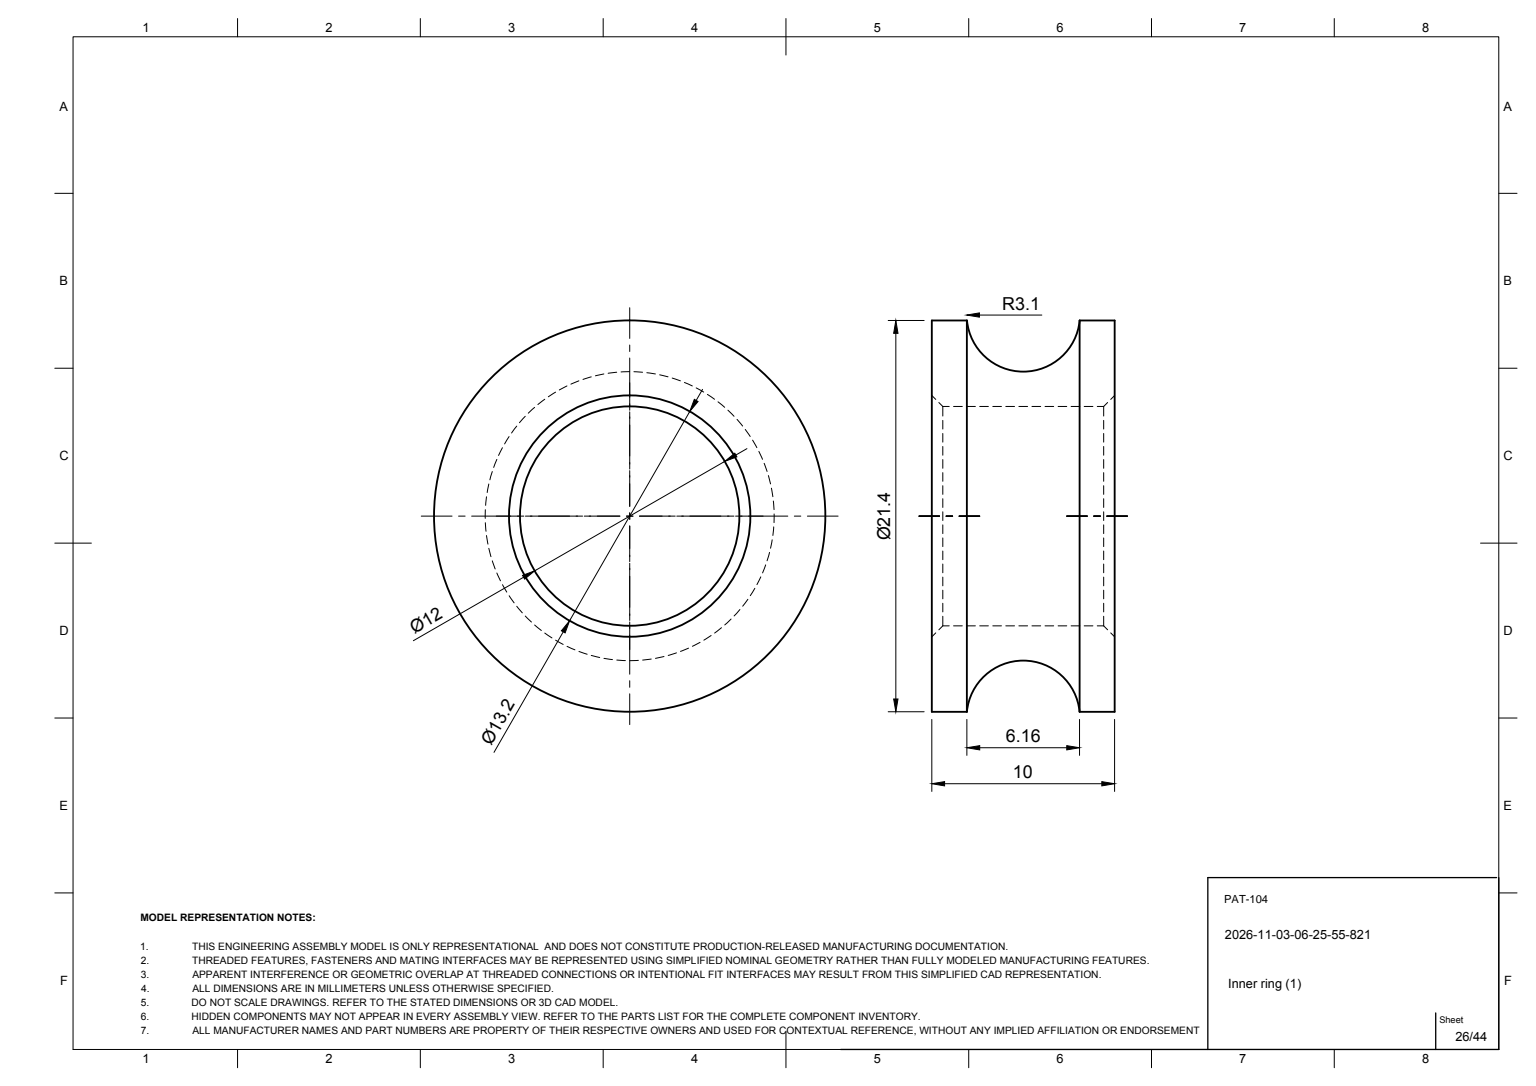
ISO-10303-21;
HEADER;
/* Generated by software containing ST-Developer
 * from STEP Tools, Inc. (www.steptools.com) 
 */

FILE_DESCRIPTION(
/* description */ ('Timing belt drive module 2 mm Pitch Timing 20T-40T'),

/* implementation_level */ '2;1');

FILE_NAME(
/* name */ 'Inner ring (1).step',
/* time_stamp */ '2026-10-28T03:25:12-07:00',
/* author */ (''),
/* organization */ (''),
/* preprocessor_version */ 'ST-DEVELOPER v20.2',
/* originating_system */ 'Autodesk Translation Framework v15.17.0.0',
/* authorisation */ '');

FILE_SCHEMA (('AUTOMOTIVE_DESIGN { 1 0 10303 214 3 1 1 }'));
ENDSEC;

DATA;
#10=MECHANICAL_DESIGN_GEOMETRIC_PRESENTATION_REPRESENTATION('',(#554),#17830);
#423=CONICAL_SURFACE('',#10053,0.63,0.785398163397448);
#424=CONICAL_SURFACE('',#10060,0.63,0.785398163397448);
#436=TOROIDAL_SURFACE('',#10042,1.1,0.309556);
#460=SHAPE_REPRESENTATION_RELATIONSHIP('SRR','None',#18032,#503);
#503=ADVANCED_BREP_SHAPE_REPRESENTATION('',(#611),#17807);
#554=STYLED_ITEM('',(#18317),#611);
#611=MANIFOLD_SOLID_BREP('Body1',#9012);
#720=FACE_BOUND('',#1807,.T.);
#721=FACE_BOUND('',#1810,.T.);
#882=PLANE('',#10055);
#883=PLANE('',#10058);
#1198=FACE_OUTER_BOUND('',#1802,.T.);
#1199=FACE_OUTER_BOUND('',#1803,.T.);
#1200=FACE_OUTER_BOUND('',#1804,.T.);
#1201=FACE_OUTER_BOUND('',#1805,.T.);
#1202=FACE_OUTER_BOUND('',#1806,.T.);
#1203=FACE_OUTER_BOUND('',#1808,.T.);
#1204=FACE_OUTER_BOUND('',#1809,.T.);
#1205=FACE_OUTER_BOUND('',#1811,.T.);
#1802=EDGE_LOOP('',(#6823,#6824,#6825,#6826,#6827,#6828));
#1803=EDGE_LOOP('',(#6829,#6830,#6831,#6832,#6833));
#1804=EDGE_LOOP('',(#6834,#6835,#6836,#6837));
#1805=EDGE_LOOP('',(#6838,#6839,#6840,#6841));
#1806=EDGE_LOOP('',(#6842));
#1807=EDGE_LOOP('',(#6843));
#1808=EDGE_LOOP('',(#6844,#6845,#6846,#6847,#6848));
#1809=EDGE_LOOP('',(#6849));
#1810=EDGE_LOOP('',(#6850));
#1811=EDGE_LOOP('',(#6851,#6852,#6853,#6854));
#2398=CIRCLE('',#10043,1.070235);
#2399=CIRCLE('',#10044,1.070235);
#2400=CIRCLE('',#10045,0.309556);
#2401=CIRCLE('',#10046,1.070235);
#2402=CIRCLE('',#10047,1.070235);
#2403=CIRCLE('',#10049,1.070235);
#2404=CIRCLE('',#10051,0.6);
#2405=CIRCLE('',#10052,0.6);
#2406=CIRCLE('',#10054,0.66);
#2407=CIRCLE('',#10057,1.070235);
#2408=CIRCLE('',#10059,0.66);
#3039=LINE('',#15374,#3517);
#3040=LINE('',#15380,#3518);
#3041=LINE('',#15384,#3519);
#3042=LINE('',#15390,#3520);
#3043=LINE('',#15395,#3521);
#3517=VECTOR('',#12124,1.070235);
#3518=VECTOR('',#12131,0.6);
#3519=VECTOR('',#12136,0.63);
#3520=VECTOR('',#12145,1.070235);
#3521=VECTOR('',#12152,0.63);
#4104=VERTEX_POINT('',#15363);
#4105=VERTEX_POINT('',#15364);
#4106=VERTEX_POINT('',#15367);
#4107=VERTEX_POINT('',#15369);
#4108=VERTEX_POINT('',#15373);
#4109=VERTEX_POINT('',#15377);
#4110=VERTEX_POINT('',#15379);
#4111=VERTEX_POINT('',#15383);
#4112=VERTEX_POINT('',#15388);
#4113=VERTEX_POINT('',#15392);
#5094=EDGE_CURVE('',#4104,#4105,#2398,.T.);
#5095=EDGE_CURVE('',#4105,#4104,#2399,.T.);
#5096=EDGE_CURVE('',#4105,#4106,#2400,.T.);
#5097=EDGE_CURVE('',#4107,#4106,#2401,.T.);
#5098=EDGE_CURVE('',#4106,#4107,#2402,.T.);
#5099=EDGE_CURVE('',#4107,#4108,#3039,.T.);
#5100=EDGE_CURVE('',#4108,#4108,#2403,.T.);
#5101=EDGE_CURVE('',#4109,#4109,#2404,.T.);
#5102=EDGE_CURVE('',#4109,#4110,#3040,.T.);
#5103=EDGE_CURVE('',#4110,#4110,#2405,.T.);
#5104=EDGE_CURVE('',#4110,#4111,#3041,.T.);
#5105=EDGE_CURVE('',#4111,#4111,#2406,.T.);
#5106=EDGE_CURVE('',#4112,#4112,#2407,.T.);
#5107=EDGE_CURVE('',#4112,#4104,#3042,.T.);
#5108=EDGE_CURVE('',#4113,#4113,#2408,.T.);
#5109=EDGE_CURVE('',#4113,#4109,#3043,.T.);
#6823=ORIENTED_EDGE('',*,*,#5094,.F.);
#6824=ORIENTED_EDGE('',*,*,#5095,.F.);
#6825=ORIENTED_EDGE('',*,*,#5096,.T.);
#6826=ORIENTED_EDGE('',*,*,#5097,.F.);
#6827=ORIENTED_EDGE('',*,*,#5098,.F.);
#6828=ORIENTED_EDGE('',*,*,#5096,.F.);
#6829=ORIENTED_EDGE('',*,*,#5097,.T.);
#6830=ORIENTED_EDGE('',*,*,#5098,.T.);
#6831=ORIENTED_EDGE('',*,*,#5099,.T.);
#6832=ORIENTED_EDGE('',*,*,#5100,.T.);
#6833=ORIENTED_EDGE('',*,*,#5099,.F.);
#6834=ORIENTED_EDGE('',*,*,#5101,.T.);
#6835=ORIENTED_EDGE('',*,*,#5102,.T.);
#6836=ORIENTED_EDGE('',*,*,#5103,.F.);
#6837=ORIENTED_EDGE('',*,*,#5102,.F.);
#6838=ORIENTED_EDGE('',*,*,#5103,.T.);
#6839=ORIENTED_EDGE('',*,*,#5104,.T.);
#6840=ORIENTED_EDGE('',*,*,#5105,.F.);
#6841=ORIENTED_EDGE('',*,*,#5104,.F.);
#6842=ORIENTED_EDGE('',*,*,#5100,.F.);
#6843=ORIENTED_EDGE('',*,*,#5105,.T.);
#6844=ORIENTED_EDGE('',*,*,#5106,.F.);
#6845=ORIENTED_EDGE('',*,*,#5107,.T.);
#6846=ORIENTED_EDGE('',*,*,#5094,.T.);
#6847=ORIENTED_EDGE('',*,*,#5095,.T.);
#6848=ORIENTED_EDGE('',*,*,#5107,.F.);
#6849=ORIENTED_EDGE('',*,*,#5106,.T.);
#6850=ORIENTED_EDGE('',*,*,#5108,.F.);
#6851=ORIENTED_EDGE('',*,*,#5108,.T.);
#6852=ORIENTED_EDGE('',*,*,#5109,.T.);
#6853=ORIENTED_EDGE('',*,*,#5101,.F.);
#6854=ORIENTED_EDGE('',*,*,#5109,.F.);
#8282=CYLINDRICAL_SURFACE('',#10048,1.070235);
#8283=CYLINDRICAL_SURFACE('',#10050,0.6);
#8284=CYLINDRICAL_SURFACE('',#10056,1.070235);
#8696=ADVANCED_FACE('',(#1198),#436,.F.);
#8697=ADVANCED_FACE('',(#1199),#8282,.T.);
#8698=ADVANCED_FACE('',(#1200),#8283,.F.);
#8699=ADVANCED_FACE('',(#1201),#423,.F.);
#8700=ADVANCED_FACE('',(#1202,#720),#882,.T.);
#8701=ADVANCED_FACE('',(#1203),#8284,.T.);
#8702=ADVANCED_FACE('',(#1204,#721),#883,.T.);
#8703=ADVANCED_FACE('',(#1205),#424,.F.);
#9012=CLOSED_SHELL('',(#8696,#8697,#8698,#8699,#8700,#8701,#8702,#8703));
#10041=AXIS2_PLACEMENT_3D('',#15361,#12108,#12109);
#10042=AXIS2_PLACEMENT_3D('',#15362,#12110,#12111);
#10043=AXIS2_PLACEMENT_3D('',#15365,#12112,#12113);
#10044=AXIS2_PLACEMENT_3D('',#15366,#12114,#12115);
#10045=AXIS2_PLACEMENT_3D('',#15368,#12116,#12117);
#10046=AXIS2_PLACEMENT_3D('',#15370,#12118,#12119);
#10047=AXIS2_PLACEMENT_3D('',#15371,#12120,#12121);
#10048=AXIS2_PLACEMENT_3D('',#15372,#12122,#12123);
#10049=AXIS2_PLACEMENT_3D('',#15375,#12125,#12126);
#10050=AXIS2_PLACEMENT_3D('',#15376,#12127,#12128);
#10051=AXIS2_PLACEMENT_3D('',#15378,#12129,#12130);
#10052=AXIS2_PLACEMENT_3D('',#15381,#12132,#12133);
#10053=AXIS2_PLACEMENT_3D('',#15382,#12134,#12135);
#10054=AXIS2_PLACEMENT_3D('',#15385,#12137,#12138);
#10055=AXIS2_PLACEMENT_3D('',#15386,#12139,#12140);
#10056=AXIS2_PLACEMENT_3D('',#15387,#12141,#12142);
#10057=AXIS2_PLACEMENT_3D('',#15389,#12143,#12144);
#10058=AXIS2_PLACEMENT_3D('',#15391,#12146,#12147);
#10059=AXIS2_PLACEMENT_3D('',#15393,#12148,#12149);
#10060=AXIS2_PLACEMENT_3D('',#15394,#12150,#12151);
#12108=DIRECTION('axis',(0.,0.,1.));
#12109=DIRECTION('refdir',(1.,0.,0.));
#12110=DIRECTION('center_axis',(0.,-1.,0.));
#12111=DIRECTION('ref_axis',(0.,0.,-1.));
#12112=DIRECTION('center_axis',(0.,-1.,0.));
#12113=DIRECTION('ref_axis',(1.,0.,0.));
#12114=DIRECTION('center_axis',(0.,-1.,0.));
#12115=DIRECTION('ref_axis',(1.,0.,0.));
#12116=DIRECTION('center_axis',(1.,0.,1.22464679914735E-16));
#12117=DIRECTION('ref_axis',(-1.22464679914735E-16,0.,1.));
#12118=DIRECTION('center_axis',(0.,1.,0.));
#12119=DIRECTION('ref_axis',(1.,0.,0.));
#12120=DIRECTION('center_axis',(0.,1.,0.));
#12121=DIRECTION('ref_axis',(1.,0.,0.));
#12122=DIRECTION('center_axis',(0.,-1.,0.));
#12123=DIRECTION('ref_axis',(1.,0.,0.));
#12124=DIRECTION('',(0.,1.,0.));
#12125=DIRECTION('center_axis',(0.,-1.,0.));
#12126=DIRECTION('ref_axis',(1.,0.,0.));
#12127=DIRECTION('center_axis',(0.,-1.,0.));
#12128=DIRECTION('ref_axis',(1.,0.,0.));
#12129=DIRECTION('center_axis',(0.,-1.,0.));
#12130=DIRECTION('ref_axis',(1.,0.,0.));
#12131=DIRECTION('',(0.,1.,0.));
#12132=DIRECTION('center_axis',(0.,-1.,0.));
#12133=DIRECTION('ref_axis',(1.,0.,0.));
#12134=DIRECTION('center_axis',(0.,1.,0.));
#12135=DIRECTION('ref_axis',(1.,0.,0.));
#12136=DIRECTION('',(-0.707106781186548,0.707106781186547,-8.65956056235493E-17));
#12137=DIRECTION('center_axis',(0.,-1.,0.));
#12138=DIRECTION('ref_axis',(1.,0.,0.));
#12139=DIRECTION('center_axis',(0.,1.,0.));
#12140=DIRECTION('ref_axis',(0.,0.,1.));
#12141=DIRECTION('center_axis',(0.,-1.,0.));
#12142=DIRECTION('ref_axis',(1.,0.,0.));
#12143=DIRECTION('center_axis',(0.,-1.,0.));
#12144=DIRECTION('ref_axis',(1.,0.,0.));
#12145=DIRECTION('',(0.,1.,0.));
#12146=DIRECTION('center_axis',(0.,-1.,0.));
#12147=DIRECTION('ref_axis',(0.,0.,-1.));
#12148=DIRECTION('center_axis',(0.,-1.,0.));
#12149=DIRECTION('ref_axis',(1.,0.,0.));
#12150=DIRECTION('center_axis',(0.,-1.,0.));
#12151=DIRECTION('ref_axis',(1.,0.,0.));
#12152=DIRECTION('',(0.707106781186548,0.707106781186547,8.65956056235493E-17));
#15361=CARTESIAN_POINT('',(0.,0.,0.));
#15362=CARTESIAN_POINT('Origin',(0.,0.,0.));
#15363=CARTESIAN_POINT('',(-1.070235,-0.308121667383195,-1.31065986708547E-16));
#15364=CARTESIAN_POINT('',(-1.31065986708547E-16,-0.308121667383195,1.070235));
#15365=CARTESIAN_POINT('Origin',(0.,-0.308121667383195,0.));
#15366=CARTESIAN_POINT('Origin',(0.,-0.308121667383195,0.));
#15367=CARTESIAN_POINT('',(-1.31065986708547E-16,0.308121667383195,1.070235));
#15368=CARTESIAN_POINT('Origin',(-1.34711147906209E-16,0.,1.1));
#15369=CARTESIAN_POINT('',(-1.070235,0.308121667383195,1.31065986708547E-16));
#15370=CARTESIAN_POINT('Origin',(0.,0.308121667383195,0.));
#15371=CARTESIAN_POINT('Origin',(0.,0.308121667383195,0.));
#15372=CARTESIAN_POINT('Origin',(0.,0.,0.));
#15373=CARTESIAN_POINT('',(-1.070235,0.5,-1.31065986708547E-16));
#15374=CARTESIAN_POINT('',(-1.070235,0.,-1.31065986708547E-16));
#15375=CARTESIAN_POINT('Origin',(0.,0.5,0.));
#15376=CARTESIAN_POINT('Origin',(0.,0.,0.));
#15377=CARTESIAN_POINT('',(-0.6,-0.44,-7.34788079488412E-17));
#15378=CARTESIAN_POINT('Origin',(0.,-0.44,0.));
#15379=CARTESIAN_POINT('',(-0.6,0.44,-7.34788079488412E-17));
#15380=CARTESIAN_POINT('',(-0.6,0.,-7.34788079488412E-17));
#15381=CARTESIAN_POINT('Origin',(0.,0.44,0.));
#15382=CARTESIAN_POINT('Origin',(0.,0.47,0.));
#15383=CARTESIAN_POINT('',(-0.66,0.5,-8.08266887437253E-17));
#15384=CARTESIAN_POINT('',(-0.63,0.47,-7.71527483462832E-17));
#15385=CARTESIAN_POINT('Origin',(0.,0.5,0.));
#15386=CARTESIAN_POINT('Origin',(1.070235,0.5,0.));
#15387=CARTESIAN_POINT('Origin',(0.,0.,0.));
#15388=CARTESIAN_POINT('',(-1.070235,-0.5,-1.31065986708547E-16));
#15389=CARTESIAN_POINT('Origin',(0.,-0.5,0.));
#15390=CARTESIAN_POINT('',(-1.070235,0.,-1.31065986708547E-16));
#15391=CARTESIAN_POINT('Origin',(0.66,-0.5,0.));
#15392=CARTESIAN_POINT('',(-0.66,-0.5,-8.08266887437253E-17));
#15393=CARTESIAN_POINT('Origin',(0.,-0.5,0.));
#15394=CARTESIAN_POINT('Origin',(0.,-0.47,0.));
#15395=CARTESIAN_POINT('',(-0.63,-0.47,-7.71527483462832E-17));
#17757=UNCERTAINTY_MEASURE_WITH_UNIT(LENGTH_MEASURE(0.001),#17831,
'DISTANCE_ACCURACY_VALUE',
'Maximum model space distance between geometric entities at asserted c
onnectivities');
#17780=UNCERTAINTY_MEASURE_WITH_UNIT(LENGTH_MEASURE(0.001),#17831,
'DISTANCE_ACCURACY_VALUE',
'Maximum model space distance between geometric entities at asserted c
onnectivities');
#17807=(
GEOMETRIC_REPRESENTATION_CONTEXT(3)
GLOBAL_UNCERTAINTY_ASSIGNED_CONTEXT((#17757))
GLOBAL_UNIT_ASSIGNED_CONTEXT((#17831,#17833,#17834))
REPRESENTATION_CONTEXT('','3D')
);
#17830=(
GEOMETRIC_REPRESENTATION_CONTEXT(3)
GLOBAL_UNCERTAINTY_ASSIGNED_CONTEXT((#17780))
GLOBAL_UNIT_ASSIGNED_CONTEXT((#17831,#17833,#17834))
REPRESENTATION_CONTEXT('','3D')
);
#17831=(
LENGTH_UNIT()
NAMED_UNIT(*)
SI_UNIT(.CENTI.,.METRE.)
);
#17833=(
NAMED_UNIT(*)
PLANE_ANGLE_UNIT()
SI_UNIT($,.RADIAN.)
);
#17834=(
NAMED_UNIT(*)
SI_UNIT($,.STERADIAN.)
SOLID_ANGLE_UNIT()
);
#17861=SHAPE_DEFINITION_REPRESENTATION(#17915,#18032);
#17915=PRODUCT_DEFINITION_SHAPE('',$,#18082);
#18032=SHAPE_REPRESENTATION('',(#10041),#17807);
#18055=PRODUCT_DEFINITION_CONTEXT('part definition',#18204,'design');
#18082=PRODUCT_DEFINITION('Inner ring (1)','Inner ring (1)',#18131,#18055);
#18131=PRODUCT_DEFINITION_FORMATION('',$,#18232);
#18204=APPLICATION_CONTEXT(
'Core Data for Automotive Mechanical Design Process');
#18205=PRODUCT_CONTEXT('part definition',#18204,'mechanical');
#18232=PRODUCT('Inner ring (1)','Inner ring (1)','Inner ring (1)',(#18205));
#18311=COLOUR_RGB('Grey',0.48,0.52,0.57);
#18312=FILL_AREA_STYLE_COLOUR('',#18311);
#18313=FILL_AREA_STYLE('',(#18312));
#18314=SURFACE_STYLE_FILL_AREA(#18313);
#18315=SURFACE_SIDE_STYLE('',(#18314));
#18316=SURFACE_STYLE_USAGE(.BOTH.,#18315);
#18317=PRESENTATION_STYLE_ASSIGNMENT((#18316));
ENDSEC;
END-ISO-10303-21;
